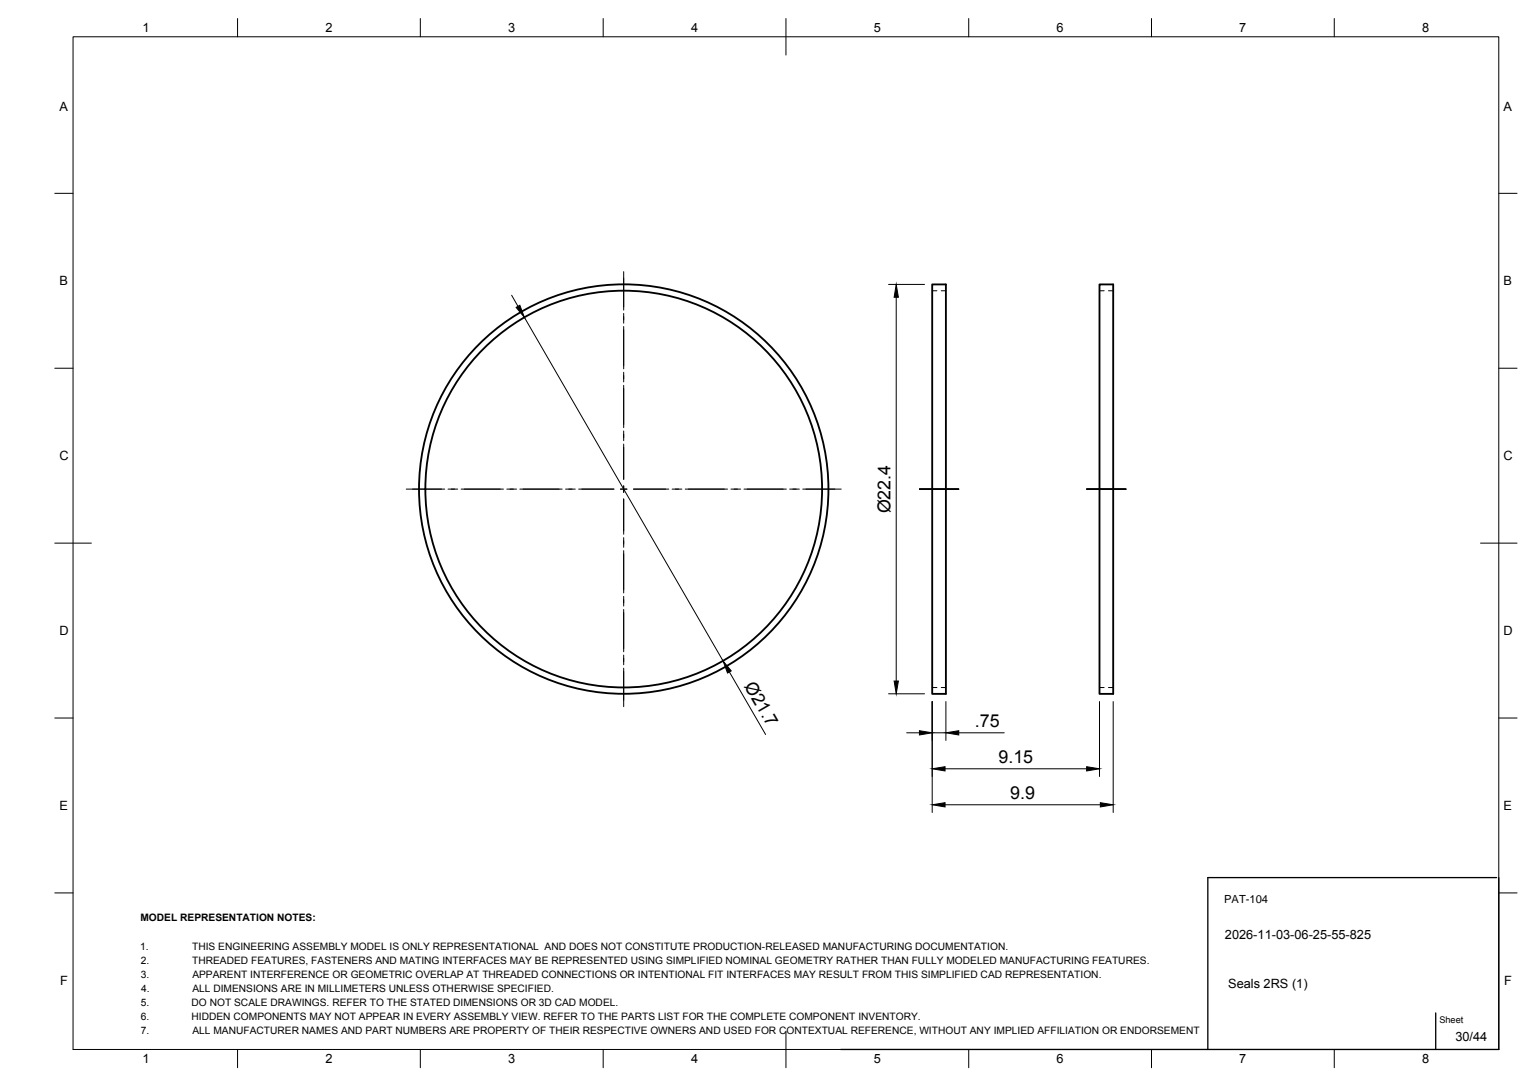
ISO-10303-21;
HEADER;
/* Generated by software containing ST-Developer
 * from STEP Tools, Inc. (www.steptools.com) 
 */

FILE_DESCRIPTION(
/* description */ ('Timing belt drive module 2 mm Pitch Timing 20T-40T'),

/* implementation_level */ '2;1');

FILE_NAME(
/* name */ 'Seals 2RS (1).step',
/* time_stamp */ '2026-10-28T03:25:12-07:00',
/* author */ (''),
/* organization */ (''),
/* preprocessor_version */ 'ST-DEVELOPER v20.2',
/* originating_system */ 'Autodesk Translation Framework v15.17.0.0',
/* authorisation */ '');

FILE_SCHEMA (('AUTOMOTIVE_DESIGN { 1 0 10303 214 3 1 1 }'));
ENDSEC;

DATA;
#10=MECHANICAL_DESIGN_GEOMETRIC_PRESENTATION_REPRESENTATION('',(#564,#565),#17830);
#464=SHAPE_REPRESENTATION_RELATIONSHIP('SRR','None',#18036,#507);
#507=ADVANCED_BREP_SHAPE_REPRESENTATION('',(#621,#622),#17811);
#564=STYLED_ITEM('',(#18317),#621);
#565=STYLED_ITEM('',(#18317),#622);
#621=MANIFOLD_SOLID_BREP('Body1',#9022);
#622=MANIFOLD_SOLID_BREP('Body2',#9023);
#725=FACE_BOUND('',#1848,.T.);
#726=FACE_BOUND('',#1851,.T.);
#727=FACE_BOUND('',#1854,.T.);
#728=FACE_BOUND('',#1857,.T.);
#894=PLANE('',#10147);
#895=PLANE('',#10152);
#896=PLANE('',#10155);
#897=PLANE('',#10160);
#1238=FACE_OUTER_BOUND('',#1847,.T.);
#1239=FACE_OUTER_BOUND('',#1849,.T.);
#1240=FACE_OUTER_BOUND('',#1850,.T.);
#1241=FACE_OUTER_BOUND('',#1852,.T.);
#1242=FACE_OUTER_BOUND('',#1853,.T.);
#1243=FACE_OUTER_BOUND('',#1855,.T.);
#1244=FACE_OUTER_BOUND('',#1856,.T.);
#1245=FACE_OUTER_BOUND('',#1858,.T.);
#1847=EDGE_LOOP('',(#6997));
#1848=EDGE_LOOP('',(#6998));
#1849=EDGE_LOOP('',(#6999,#7000,#7001,#7002));
#1850=EDGE_LOOP('',(#7003));
#1851=EDGE_LOOP('',(#7004));
#1852=EDGE_LOOP('',(#7005,#7006,#7007,#7008));
#1853=EDGE_LOOP('',(#7009));
#1854=EDGE_LOOP('',(#7010));
#1855=EDGE_LOOP('',(#7011,#7012,#7013,#7014));
#1856=EDGE_LOOP('',(#7015));
#1857=EDGE_LOOP('',(#7016));
#1858=EDGE_LOOP('',(#7017,#7018,#7019,#7020));
#2459=CIRCLE('',#10148,1.119765);
#2460=CIRCLE('',#10149,1.085235);
#2461=CIRCLE('',#10151,1.119765);
#2462=CIRCLE('',#10153,1.085235);
#2463=CIRCLE('',#10156,1.119765);
#2464=CIRCLE('',#10157,1.085235);
#2465=CIRCLE('',#10159,1.119765);
#2466=CIRCLE('',#10161,1.085235);
#3051=LINE('',#15861,#3529);
#3052=LINE('',#15866,#3530);
#3053=LINE('',#15875,#3531);
#3054=LINE('',#15880,#3532);
#3529=VECTOR('',#12342,1.119765);
#3530=VECTOR('',#12349,1.085235);
#3531=VECTOR('',#12360,1.119765);
#3532=VECTOR('',#12367,1.085235);
#4170=VERTEX_POINT('',#15854);
#4171=VERTEX_POINT('',#15856);
#4172=VERTEX_POINT('',#15859);
#4173=VERTEX_POINT('',#15863);
#4174=VERTEX_POINT('',#15868);
#4175=VERTEX_POINT('',#15870);
#4176=VERTEX_POINT('',#15873);
#4177=VERTEX_POINT('',#15877);
#5181=EDGE_CURVE('',#4170,#4170,#2459,.T.);
#5182=EDGE_CURVE('',#4171,#4171,#2460,.T.);
#5183=EDGE_CURVE('',#4172,#4172,#2461,.T.);
#5184=EDGE_CURVE('',#4172,#4170,#3051,.T.);
#5185=EDGE_CURVE('',#4173,#4173,#2462,.T.);
#5186=EDGE_CURVE('',#4173,#4171,#3052,.T.);
#5187=EDGE_CURVE('',#4174,#4174,#2463,.T.);
#5188=EDGE_CURVE('',#4175,#4175,#2464,.T.);
#5189=EDGE_CURVE('',#4176,#4176,#2465,.T.);
#5190=EDGE_CURVE('',#4176,#4174,#3053,.T.);
#5191=EDGE_CURVE('',#4177,#4177,#2466,.T.);
#5192=EDGE_CURVE('',#4177,#4175,#3054,.T.);
#6997=ORIENTED_EDGE('',*,*,#5181,.F.);
#6998=ORIENTED_EDGE('',*,*,#5182,.T.);
#6999=ORIENTED_EDGE('',*,*,#5183,.F.);
#7000=ORIENTED_EDGE('',*,*,#5184,.T.);
#7001=ORIENTED_EDGE('',*,*,#5181,.T.);
#7002=ORIENTED_EDGE('',*,*,#5184,.F.);
#7003=ORIENTED_EDGE('',*,*,#5183,.T.);
#7004=ORIENTED_EDGE('',*,*,#5185,.F.);
#7005=ORIENTED_EDGE('',*,*,#5185,.T.);
#7006=ORIENTED_EDGE('',*,*,#5186,.T.);
#7007=ORIENTED_EDGE('',*,*,#5182,.F.);
#7008=ORIENTED_EDGE('',*,*,#5186,.F.);
#7009=ORIENTED_EDGE('',*,*,#5187,.F.);
#7010=ORIENTED_EDGE('',*,*,#5188,.T.);
#7011=ORIENTED_EDGE('',*,*,#5189,.F.);
#7012=ORIENTED_EDGE('',*,*,#5190,.T.);
#7013=ORIENTED_EDGE('',*,*,#5187,.T.);
#7014=ORIENTED_EDGE('',*,*,#5190,.F.);
#7015=ORIENTED_EDGE('',*,*,#5189,.T.);
#7016=ORIENTED_EDGE('',*,*,#5191,.F.);
#7017=ORIENTED_EDGE('',*,*,#5191,.T.);
#7018=ORIENTED_EDGE('',*,*,#5192,.T.);
#7019=ORIENTED_EDGE('',*,*,#5188,.F.);
#7020=ORIENTED_EDGE('',*,*,#5192,.F.);
#8290=CYLINDRICAL_SURFACE('',#10150,1.119765);
#8291=CYLINDRICAL_SURFACE('',#10154,1.085235);
#8292=CYLINDRICAL_SURFACE('',#10158,1.119765);
#8293=CYLINDRICAL_SURFACE('',#10162,1.085235);
#8736=ADVANCED_FACE('',(#1238,#725),#894,.T.);
#8737=ADVANCED_FACE('',(#1239),#8290,.T.);
#8738=ADVANCED_FACE('',(#1240,#726),#895,.T.);
#8739=ADVANCED_FACE('',(#1241),#8291,.F.);
#8740=ADVANCED_FACE('',(#1242,#727),#896,.T.);
#8741=ADVANCED_FACE('',(#1243),#8292,.T.);
#8742=ADVANCED_FACE('',(#1244,#728),#897,.T.);
#8743=ADVANCED_FACE('',(#1245),#8293,.F.);
#9022=CLOSED_SHELL('',(#8736,#8737,#8738,#8739));
#9023=CLOSED_SHELL('',(#8740,#8741,#8742,#8743));
#10146=AXIS2_PLACEMENT_3D('',#15852,#12330,#12331);
#10147=AXIS2_PLACEMENT_3D('',#15853,#12332,#12333);
#10148=AXIS2_PLACEMENT_3D('',#15855,#12334,#12335);
#10149=AXIS2_PLACEMENT_3D('',#15857,#12336,#12337);
#10150=AXIS2_PLACEMENT_3D('',#15858,#12338,#12339);
#10151=AXIS2_PLACEMENT_3D('',#15860,#12340,#12341);
#10152=AXIS2_PLACEMENT_3D('',#15862,#12343,#12344);
#10153=AXIS2_PLACEMENT_3D('',#15864,#12345,#12346);
#10154=AXIS2_PLACEMENT_3D('',#15865,#12347,#12348);
#10155=AXIS2_PLACEMENT_3D('',#15867,#12350,#12351);
#10156=AXIS2_PLACEMENT_3D('',#15869,#12352,#12353);
#10157=AXIS2_PLACEMENT_3D('',#15871,#12354,#12355);
#10158=AXIS2_PLACEMENT_3D('',#15872,#12356,#12357);
#10159=AXIS2_PLACEMENT_3D('',#15874,#12358,#12359);
#10160=AXIS2_PLACEMENT_3D('',#15876,#12361,#12362);
#10161=AXIS2_PLACEMENT_3D('',#15878,#12363,#12364);
#10162=AXIS2_PLACEMENT_3D('',#15879,#12365,#12366);
#12330=DIRECTION('axis',(0.,0.,1.));
#12331=DIRECTION('refdir',(1.,0.,0.));
#12332=DIRECTION('center_axis',(0.,1.,0.));
#12333=DIRECTION('ref_axis',(0.,0.,1.));
#12334=DIRECTION('center_axis',(0.,-1.,0.));
#12335=DIRECTION('ref_axis',(1.,0.,0.));
#12336=DIRECTION('center_axis',(0.,-1.,0.));
#12337=DIRECTION('ref_axis',(1.,0.,0.));
#12338=DIRECTION('center_axis',(0.,-1.,0.));
#12339=DIRECTION('ref_axis',(1.,0.,0.));
#12340=DIRECTION('center_axis',(0.,-1.,0.));
#12341=DIRECTION('ref_axis',(1.,0.,0.));
#12342=DIRECTION('',(0.,1.,0.));
#12343=DIRECTION('center_axis',(0.,-1.,0.));
#12344=DIRECTION('ref_axis',(0.,0.,-1.));
#12345=DIRECTION('center_axis',(0.,-1.,0.));
#12346=DIRECTION('ref_axis',(1.,0.,0.));
#12347=DIRECTION('center_axis',(0.,-1.,0.));
#12348=DIRECTION('ref_axis',(1.,0.,0.));
#12349=DIRECTION('',(0.,1.,0.));
#12350=DIRECTION('center_axis',(0.,1.,0.));
#12351=DIRECTION('ref_axis',(0.,0.,1.));
#12352=DIRECTION('center_axis',(0.,-1.,0.));
#12353=DIRECTION('ref_axis',(1.,0.,0.));
#12354=DIRECTION('center_axis',(0.,-1.,0.));
#12355=DIRECTION('ref_axis',(1.,0.,0.));
#12356=DIRECTION('center_axis',(0.,-1.,0.));
#12357=DIRECTION('ref_axis',(1.,0.,0.));
#12358=DIRECTION('center_axis',(0.,-1.,0.));
#12359=DIRECTION('ref_axis',(1.,0.,0.));
#12360=DIRECTION('',(0.,1.,0.));
#12361=DIRECTION('center_axis',(0.,-1.,0.));
#12362=DIRECTION('ref_axis',(0.,0.,-1.));
#12363=DIRECTION('center_axis',(0.,-1.,0.));
#12364=DIRECTION('ref_axis',(1.,0.,0.));
#12365=DIRECTION('center_axis',(0.,-1.,0.));
#12366=DIRECTION('ref_axis',(1.,0.,0.));
#12367=DIRECTION('',(0.,1.,0.));
#15852=CARTESIAN_POINT('',(0.,0.,0.));
#15853=CARTESIAN_POINT('Origin',(1.119765,0.495,0.));
#15854=CARTESIAN_POINT('',(-1.119765,0.495,-1.37131662304724E-16));
#15855=CARTESIAN_POINT('Origin',(0.,0.495,0.));
#15856=CARTESIAN_POINT('',(-1.085235,0.495,-1.32902956907268E-16));
#15857=CARTESIAN_POINT('Origin',(0.,0.495,0.));
#15858=CARTESIAN_POINT('Origin',(0.,0.4575,0.));
#15859=CARTESIAN_POINT('',(-1.119765,0.42,-1.37131662304724E-16));
#15860=CARTESIAN_POINT('Origin',(0.,0.42,0.));
#15861=CARTESIAN_POINT('',(-1.119765,0.4575,-1.37131662304724E-16));
#15862=CARTESIAN_POINT('Origin',(1.085235,0.42,0.));
#15863=CARTESIAN_POINT('',(-1.085235,0.42,-1.32902956907268E-16));
#15864=CARTESIAN_POINT('Origin',(0.,0.42,0.));
#15865=CARTESIAN_POINT('Origin',(0.,0.4575,0.));
#15866=CARTESIAN_POINT('',(-1.085235,0.4575,-1.32902956907268E-16));
#15867=CARTESIAN_POINT('Origin',(1.119765,-0.42,0.));
#15868=CARTESIAN_POINT('',(-1.119765,-0.42,-1.37131662304724E-16));
#15869=CARTESIAN_POINT('Origin',(0.,-0.42,0.));
#15870=CARTESIAN_POINT('',(-1.085235,-0.42,-1.32902956907268E-16));
#15871=CARTESIAN_POINT('Origin',(0.,-0.42,0.));
#15872=CARTESIAN_POINT('Origin',(0.,-0.4575,0.));
#15873=CARTESIAN_POINT('',(-1.119765,-0.495,-1.37131662304724E-16));
#15874=CARTESIAN_POINT('Origin',(0.,-0.495,0.));
#15875=CARTESIAN_POINT('',(-1.119765,-0.4575,-1.37131662304724E-16));
#15876=CARTESIAN_POINT('Origin',(1.085235,-0.495,0.));
#15877=CARTESIAN_POINT('',(-1.085235,-0.495,-1.32902956907268E-16));
#15878=CARTESIAN_POINT('Origin',(0.,-0.495,0.));
#15879=CARTESIAN_POINT('Origin',(0.,-0.4575,0.));
#15880=CARTESIAN_POINT('',(-1.085235,-0.4575,-1.32902956907268E-16));
#17761=UNCERTAINTY_MEASURE_WITH_UNIT(LENGTH_MEASURE(0.001),#17831,
'DISTANCE_ACCURACY_VALUE',
'Maximum model space distance between geometric entities at asserted c
onnectivities');
#17780=UNCERTAINTY_MEASURE_WITH_UNIT(LENGTH_MEASURE(0.001),#17831,
'DISTANCE_ACCURACY_VALUE',
'Maximum model space distance between geometric entities at asserted c
onnectivities');
#17811=(
GEOMETRIC_REPRESENTATION_CONTEXT(3)
GLOBAL_UNCERTAINTY_ASSIGNED_CONTEXT((#17761))
GLOBAL_UNIT_ASSIGNED_CONTEXT((#17831,#17833,#17834))
REPRESENTATION_CONTEXT('','3D')
);
#17830=(
GEOMETRIC_REPRESENTATION_CONTEXT(3)
GLOBAL_UNCERTAINTY_ASSIGNED_CONTEXT((#17780))
GLOBAL_UNIT_ASSIGNED_CONTEXT((#17831,#17833,#17834))
REPRESENTATION_CONTEXT('','3D')
);
#17831=(
LENGTH_UNIT()
NAMED_UNIT(*)
SI_UNIT(.CENTI.,.METRE.)
);
#17833=(
NAMED_UNIT(*)
PLANE_ANGLE_UNIT()
SI_UNIT($,.RADIAN.)
);
#17834=(
NAMED_UNIT(*)
SI_UNIT($,.STERADIAN.)
SOLID_ANGLE_UNIT()
);
#17865=SHAPE_DEFINITION_REPRESENTATION(#17919,#18036);
#17919=PRODUCT_DEFINITION_SHAPE('',$,#18086);
#18036=SHAPE_REPRESENTATION('',(#10146),#17811);
#18055=PRODUCT_DEFINITION_CONTEXT('part definition',#18204,'design');
#18086=PRODUCT_DEFINITION('Seals 2RS (1)','Seals 2RS (1)',#18135,#18055);
#18135=PRODUCT_DEFINITION_FORMATION('',$,#18236);
#18204=APPLICATION_CONTEXT(
'Core Data for Automotive Mechanical Design Process');
#18205=PRODUCT_CONTEXT('part definition',#18204,'mechanical');
#18236=PRODUCT('Seals 2RS (1)','Seals 2RS (1)','Seals 2RS (1)',(#18205));
#18311=COLOUR_RGB('Grey',0.48,0.52,0.57);
#18312=FILL_AREA_STYLE_COLOUR('',#18311);
#18313=FILL_AREA_STYLE('',(#18312));
#18314=SURFACE_STYLE_FILL_AREA(#18313);
#18315=SURFACE_SIDE_STYLE('',(#18314));
#18316=SURFACE_STYLE_USAGE(.BOTH.,#18315);
#18317=PRESENTATION_STYLE_ASSIGNMENT((#18316));
ENDSEC;
END-ISO-10303-21;
